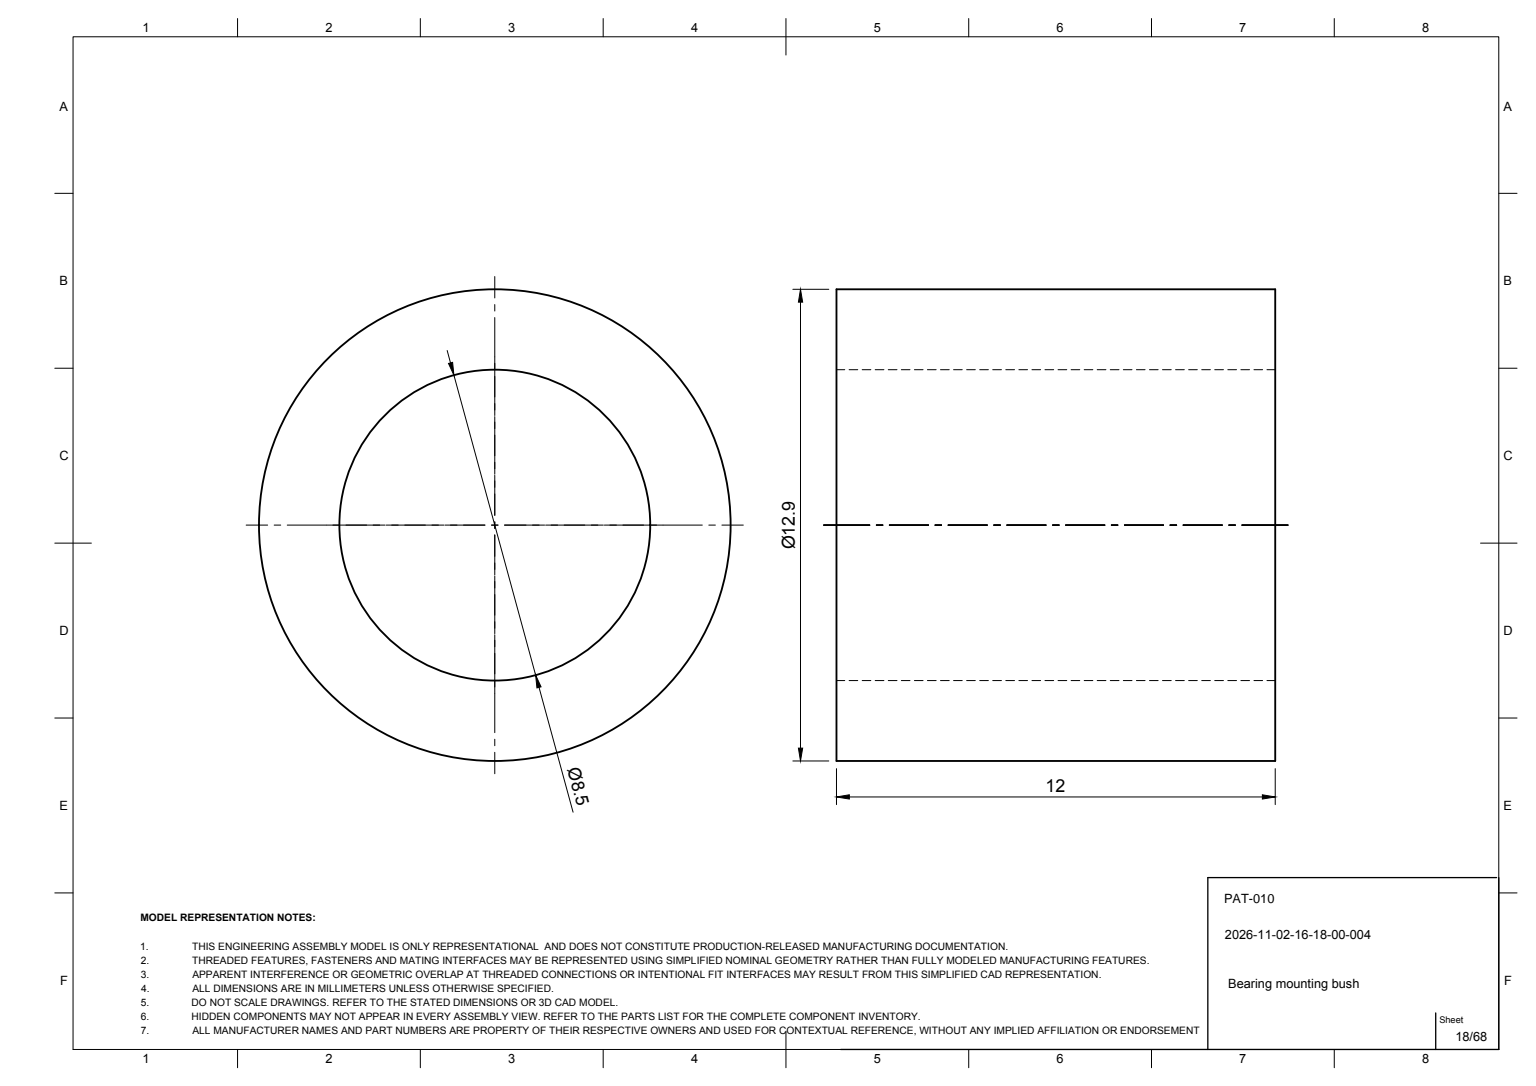
ISO-10303-21;
HEADER;
/* Generated by software containing ST-Developer
 * from STEP Tools, Inc. (www.steptools.com) 
 */

FILE_DESCRIPTION(
/* description */ ('Belt conveyor head drive unit'),
/* implementation_level */ '2;1');

FILE_NAME(
/* name */ 'Bearing mounting bush.step',
/* time_stamp */ '2026-10-28T03:26:19-07:00',
/* author */ (''),
/* organization */ (''),
/* preprocessor_version */ 'ST-DEVELOPER v20.2',
/* originating_system */ 'Autodesk Translation Framework v15.17.0.0',
/* authorisation */ '');

FILE_SCHEMA (('AUTOMOTIVE_DESIGN { 1 0 10303 214 3 1 1 }'));
ENDSEC;

DATA;
#10=MECHANICAL_DESIGN_GEOMETRIC_PRESENTATION_REPRESENTATION('',(#864),#27069);
#726=SHAPE_REPRESENTATION_RELATIONSHIP('SRR','None',#27370,#795);
#795=ADVANCED_BREP_SHAPE_REPRESENTATION('',(#949),#27012);
#864=STYLED_ITEM('',(#27797),#949);
#949=MANIFOLD_SOLID_BREP('Body1',#13729);
#1107=FACE_BOUND('',#2751,.T.);
#1108=FACE_BOUND('',#2753,.T.);
#1385=PLANE('',#15044);
#1386=PLANE('',#15045);
#1853=FACE_OUTER_BOUND('',#2748,.T.);
#1854=FACE_OUTER_BOUND('',#2749,.T.);
#1855=FACE_OUTER_BOUND('',#2750,.T.);
#1856=FACE_OUTER_BOUND('',#2752,.T.);
#2748=EDGE_LOOP('',(#9948,#9949,#9950,#9951));
#2749=EDGE_LOOP('',(#9952,#9953,#9954,#9955));
#2750=EDGE_LOOP('',(#9956));
#2751=EDGE_LOOP('',(#9957));
#2752=EDGE_LOOP('',(#9958));
#2753=EDGE_LOOP('',(#9959));
#3757=LINE('',#22039,#4549);
#3758=LINE('',#22045,#4550);
#4549=VECTOR('',#17649,0.425);
#4550=VECTOR('',#17656,0.645);
#5318=CIRCLE('',#15039,0.425);
#5319=CIRCLE('',#15040,0.425);
#5320=CIRCLE('',#15042,0.645);
#5321=CIRCLE('',#15043,0.645);
#6283=VERTEX_POINT('',#22036);
#6284=VERTEX_POINT('',#22038);
#6285=VERTEX_POINT('',#22042);
#6286=VERTEX_POINT('',#22044);
#7666=EDGE_CURVE('',#6283,#6283,#5318,.T.);
#7667=EDGE_CURVE('',#6283,#6284,#3757,.T.);
#7668=EDGE_CURVE('',#6284,#6284,#5319,.T.);
#7669=EDGE_CURVE('',#6285,#6285,#5320,.T.);
#7670=EDGE_CURVE('',#6285,#6286,#3758,.T.);
#7671=EDGE_CURVE('',#6286,#6286,#5321,.T.);
#9948=ORIENTED_EDGE('',*,*,#7666,.F.);
#9949=ORIENTED_EDGE('',*,*,#7667,.T.);
#9950=ORIENTED_EDGE('',*,*,#7668,.T.);
#9951=ORIENTED_EDGE('',*,*,#7667,.F.);
#9952=ORIENTED_EDGE('',*,*,#7669,.F.);
#9953=ORIENTED_EDGE('',*,*,#7670,.T.);
#9954=ORIENTED_EDGE('',*,*,#7671,.T.);
#9955=ORIENTED_EDGE('',*,*,#7670,.F.);
#9956=ORIENTED_EDGE('',*,*,#7669,.T.);
#9957=ORIENTED_EDGE('',*,*,#7666,.T.);
#9958=ORIENTED_EDGE('',*,*,#7671,.F.);
#9959=ORIENTED_EDGE('',*,*,#7668,.F.);
#12644=CYLINDRICAL_SURFACE('',#15038,0.425);
#12645=CYLINDRICAL_SURFACE('',#15041,0.645);
#13132=ADVANCED_FACE('',(#1853),#12644,.F.);
#13133=ADVANCED_FACE('',(#1854),#12645,.T.);
#13134=ADVANCED_FACE('',(#1855,#1107),#1385,.T.);
#13135=ADVANCED_FACE('',(#1856,#1108),#1386,.F.);
#13729=CLOSED_SHELL('',(#13132,#13133,#13134,#13135));
#15037=AXIS2_PLACEMENT_3D('',#22034,#17643,#17644);
#15038=AXIS2_PLACEMENT_3D('',#22035,#17645,#17646);
#15039=AXIS2_PLACEMENT_3D('',#22037,#17647,#17648);
#15040=AXIS2_PLACEMENT_3D('',#22040,#17650,#17651);
#15041=AXIS2_PLACEMENT_3D('',#22041,#17652,#17653);
#15042=AXIS2_PLACEMENT_3D('',#22043,#17654,#17655);
#15043=AXIS2_PLACEMENT_3D('',#22046,#17657,#17658);
#15044=AXIS2_PLACEMENT_3D('',#22047,#17659,#17660);
#15045=AXIS2_PLACEMENT_3D('',#22048,#17661,#17662);
#17643=DIRECTION('axis',(0.,0.,1.));
#17644=DIRECTION('refdir',(1.,0.,0.));
#17645=DIRECTION('center_axis',(0.,0.,1.));
#17646=DIRECTION('ref_axis',(1.,0.,0.));
#17647=DIRECTION('center_axis',(0.,0.,-1.));
#17648=DIRECTION('ref_axis',(1.,0.,0.));
#17649=DIRECTION('',(0.,0.,-1.));
#17650=DIRECTION('center_axis',(0.,0.,-1.));
#17651=DIRECTION('ref_axis',(1.,0.,0.));
#17652=DIRECTION('center_axis',(0.,0.,1.));
#17653=DIRECTION('ref_axis',(1.,0.,0.));
#17654=DIRECTION('center_axis',(0.,0.,1.));
#17655=DIRECTION('ref_axis',(1.,0.,0.));
#17656=DIRECTION('',(0.,0.,-1.));
#17657=DIRECTION('center_axis',(0.,0.,1.));
#17658=DIRECTION('ref_axis',(1.,0.,0.));
#17659=DIRECTION('center_axis',(0.,0.,1.));
#17660=DIRECTION('ref_axis',(1.,0.,0.));
#17661=DIRECTION('center_axis',(0.,0.,1.));
#17662=DIRECTION('ref_axis',(1.,0.,0.));
#22034=CARTESIAN_POINT('',(0.,0.,0.));
#22035=CARTESIAN_POINT('Origin',(2.22091003018116,4.,3.67));
#22036=CARTESIAN_POINT('',(1.79591003018116,4.,4.87));
#22037=CARTESIAN_POINT('Origin',(2.22091003018116,4.,4.87));
#22038=CARTESIAN_POINT('',(1.79591003018116,4.,3.67));
#22039=CARTESIAN_POINT('',(1.79591003018116,4.,3.67));
#22040=CARTESIAN_POINT('Origin',(2.22091003018116,4.,3.67));
#22041=CARTESIAN_POINT('Origin',(2.22091003018116,4.,3.67));
#22042=CARTESIAN_POINT('',(1.57591003018116,4.,4.87));
#22043=CARTESIAN_POINT('Origin',(2.22091003018116,4.,4.87));
#22044=CARTESIAN_POINT('',(1.57591003018116,4.,3.67));
#22045=CARTESIAN_POINT('',(1.57591003018116,4.,3.67));
#22046=CARTESIAN_POINT('Origin',(2.22091003018116,4.,3.67));
#22047=CARTESIAN_POINT('Origin',(2.22091003018116,4.,4.87));
#22048=CARTESIAN_POINT('Origin',(2.22091003018116,4.,3.67));
#26935=UNCERTAINTY_MEASURE_WITH_UNIT(LENGTH_MEASURE(0.001),#27070,
'DISTANCE_ACCURACY_VALUE',
'Maximum model space distance between geometric entities at asserted c
onnectivities');
#26992=UNCERTAINTY_MEASURE_WITH_UNIT(LENGTH_MEASURE(0.001),#27070,
'DISTANCE_ACCURACY_VALUE',
'Maximum model space distance between geometric entities at asserted c
onnectivities');
#27012=(
GEOMETRIC_REPRESENTATION_CONTEXT(3)
GLOBAL_UNCERTAINTY_ASSIGNED_CONTEXT((#26935))
GLOBAL_UNIT_ASSIGNED_CONTEXT((#27070,#27072,#27073))
REPRESENTATION_CONTEXT('','3D')
);
#27069=(
GEOMETRIC_REPRESENTATION_CONTEXT(3)
GLOBAL_UNCERTAINTY_ASSIGNED_CONTEXT((#26992))
GLOBAL_UNIT_ASSIGNED_CONTEXT((#27070,#27072,#27073))
REPRESENTATION_CONTEXT('','3D')
);
#27070=(
LENGTH_UNIT()
NAMED_UNIT(*)
SI_UNIT(.CENTI.,.METRE.)
);
#27072=(
NAMED_UNIT(*)
PLANE_ANGLE_UNIT()
SI_UNIT($,.RADIAN.)
);
#27073=(
NAMED_UNIT(*)
SI_UNIT($,.STERADIAN.)
SOLID_ANGLE_UNIT()
);
#27093=SHAPE_DEFINITION_REPRESENTATION(#27169,#27370);
#27169=PRODUCT_DEFINITION_SHAPE('',$,#27447);
#27370=SHAPE_REPRESENTATION('',(#15037),#27012);
#27427=PRODUCT_DEFINITION_CONTEXT('part definition',#27657,'design');
#27447=PRODUCT_DEFINITION('Bearing mounting bush',
'Bearing mounting bush',#27523,#27427);
#27523=PRODUCT_DEFINITION_FORMATION('',$,#27678);
#27657=APPLICATION_CONTEXT(
'Core Data for Automotive Mechanical Design Process');
#27658=PRODUCT_CONTEXT('part definition',#27657,'mechanical');
#27678=PRODUCT('Bearing mounting bush','Bearing mounting bush',
'Bearing mounting bush',(#27658));
#27791=COLOUR_RGB('Grey',0.48,0.52,0.57);
#27792=FILL_AREA_STYLE_COLOUR('',#27791);
#27793=FILL_AREA_STYLE('',(#27792));
#27794=SURFACE_STYLE_FILL_AREA(#27793);
#27795=SURFACE_SIDE_STYLE('',(#27794));
#27796=SURFACE_STYLE_USAGE(.BOTH.,#27795);
#27797=PRESENTATION_STYLE_ASSIGNMENT((#27796));
ENDSEC;
END-ISO-10303-21;
